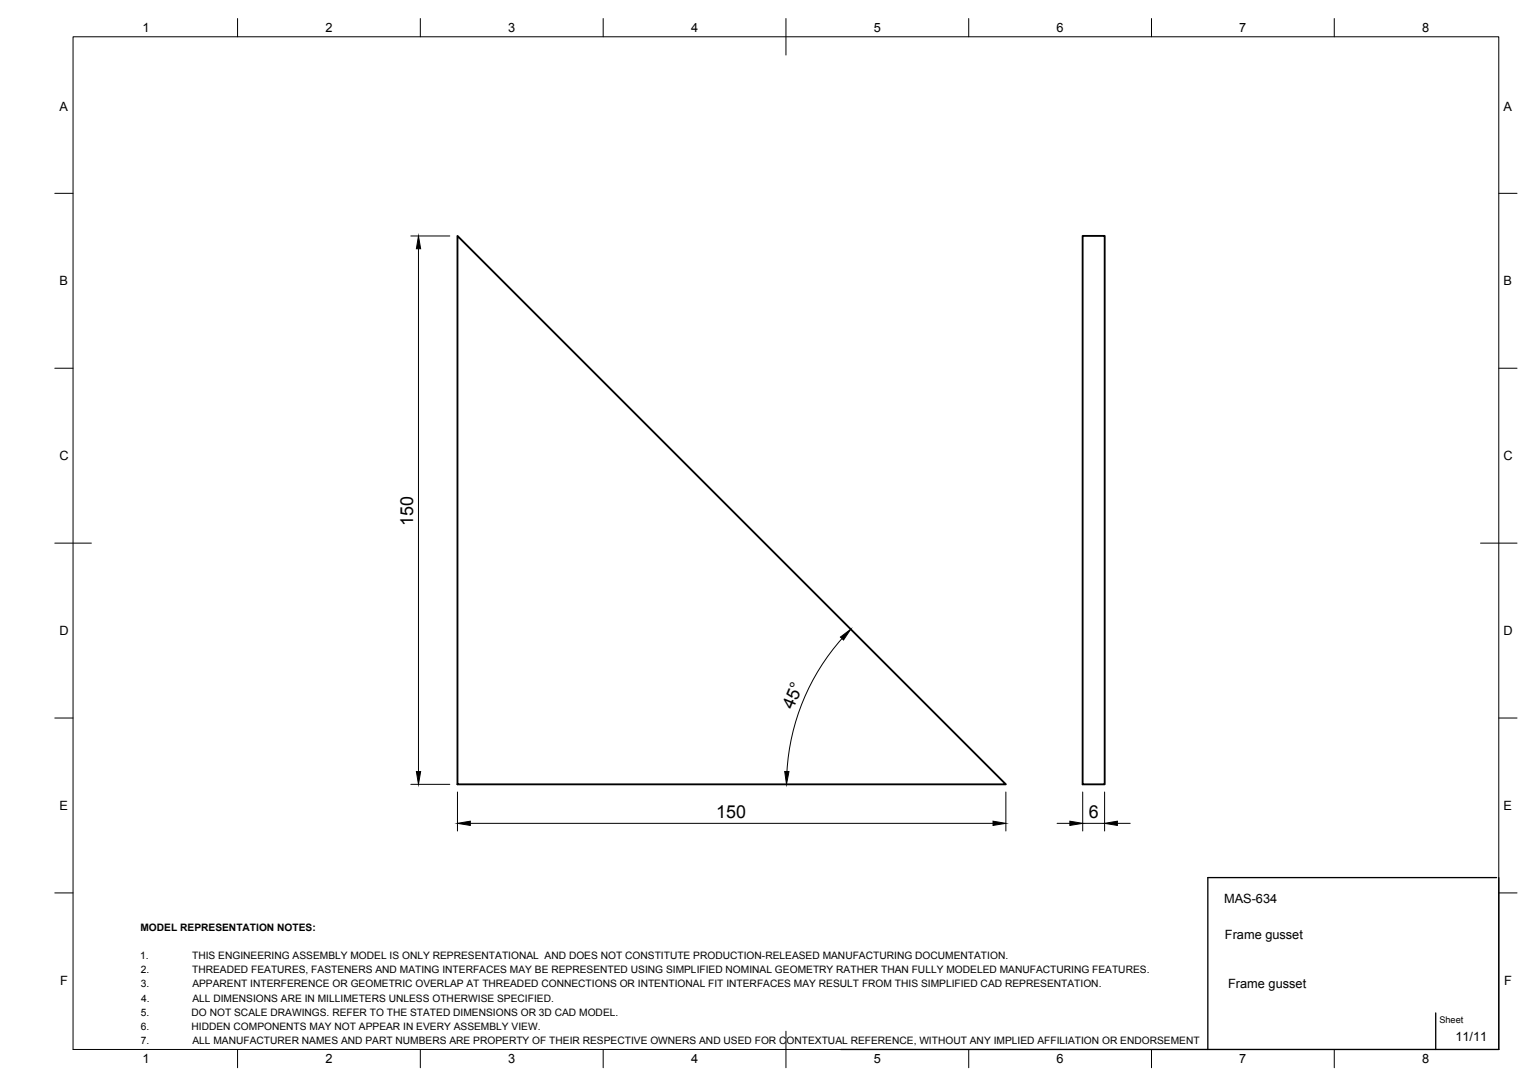
ISO-10303-21;
HEADER;
/* Generated by software containing ST-Developer
 * from STEP Tools, Inc. (www.steptools.com) 
 */

FILE_DESCRIPTION(
/* description */ ('Independent AHU equipment rack. Nominal800x600 frame on1000long40squa
re aluminum posts; two removable notched shelves; welded perimeter/cro
ss rails and rear gussets; two mounting channels; four isolation pads 
and anchor-ready feet. Imported native extrusion library retained and 
cut-length parameters customized per family. Shelf hardware uses model
ed M6 rivet nuts and screws. Weld design, floor anchors and load ratin
g require engineering selection.'),
/* implementation_level */ '2;1');

FILE_NAME(
/* name */ 'Frame gusset.step',
/* time_stamp */ '2026-11-07T19:04:45-08:00',
/* author */ (''),
/* organization */ (''),
/* preprocessor_version */ 'ST-DEVELOPER v20.2',
/* originating_system */ 'Autodesk Translation Framework v15.17.0.0',
/* authorisation */ '');

FILE_SCHEMA (('AUTOMOTIVE_DESIGN { 1 0 10303 214 3 1 1 }'));
ENDSEC;

DATA;
#10=MECHANICAL_DESIGN_GEOMETRIC_PRESENTATION_REPRESENTATION('',(#343),#9777);
#321=SHAPE_REPRESENTATION_RELATIONSHIP('SRR','None',#9865,#332);
#332=ADVANCED_BREP_SHAPE_REPRESENTATION('',(#354),#9774);
#343=STYLED_ITEM('',(#9928),#354);
#354=MANIFOLD_SOLID_BREP('Body1',#3848);
#482=PLANE('',#4211);
#483=PLANE('',#4212);
#484=PLANE('',#4213);
#485=PLANE('',#4214);
#486=PLANE('',#4215);
#626=FACE_OUTER_BOUND('',#870,.T.);
#627=FACE_OUTER_BOUND('',#871,.T.);
#628=FACE_OUTER_BOUND('',#872,.T.);
#629=FACE_OUTER_BOUND('',#873,.T.);
#630=FACE_OUTER_BOUND('',#874,.T.);
#870=EDGE_LOOP('',(#3163,#3164,#3165,#3166));
#871=EDGE_LOOP('',(#3167,#3168,#3169,#3170));
#872=EDGE_LOOP('',(#3171,#3172,#3173,#3174));
#873=EDGE_LOOP('',(#3175,#3176,#3177));
#874=EDGE_LOOP('',(#3178,#3179,#3180));
#1171=LINE('',#6080,#1464);
#1172=LINE('',#6082,#1465);
#1173=LINE('',#6084,#1466);
#1174=LINE('',#6085,#1467);
#1175=LINE('',#6088,#1468);
#1176=LINE('',#6090,#1469);
#1177=LINE('',#6091,#1470);
#1178=LINE('',#6093,#1471);
#1179=LINE('',#6094,#1472);
#1464=VECTOR('',#5050,10.);
#1465=VECTOR('',#5051,10.);
#1466=VECTOR('',#5052,10.);
#1467=VECTOR('',#5053,10.);
#1468=VECTOR('',#5056,10.);
#1469=VECTOR('',#5057,10.);
#1470=VECTOR('',#5058,10.);
#1471=VECTOR('',#5061,10.);
#1472=VECTOR('',#5062,10.);
#1876=VERTEX_POINT('',#6078);
#1877=VERTEX_POINT('',#6079);
#1878=VERTEX_POINT('',#6081);
#1879=VERTEX_POINT('',#6083);
#1880=VERTEX_POINT('',#6087);
#1881=VERTEX_POINT('',#6089);
#2326=EDGE_CURVE('',#1876,#1877,#1171,.T.);
#2327=EDGE_CURVE('',#1877,#1878,#1172,.T.);
#2328=EDGE_CURVE('',#1879,#1878,#1173,.T.);
#2329=EDGE_CURVE('',#1876,#1879,#1174,.T.);
#2330=EDGE_CURVE('',#1880,#1876,#1175,.T.);
#2331=EDGE_CURVE('',#1881,#1879,#1176,.T.);
#2332=EDGE_CURVE('',#1880,#1881,#1177,.T.);
#2333=EDGE_CURVE('',#1877,#1880,#1178,.T.);
#2334=EDGE_CURVE('',#1878,#1881,#1179,.T.);
#3163=ORIENTED_EDGE('',*,*,#2326,.T.);
#3164=ORIENTED_EDGE('',*,*,#2327,.T.);
#3165=ORIENTED_EDGE('',*,*,#2328,.F.);
#3166=ORIENTED_EDGE('',*,*,#2329,.F.);
#3167=ORIENTED_EDGE('',*,*,#2330,.T.);
#3168=ORIENTED_EDGE('',*,*,#2329,.T.);
#3169=ORIENTED_EDGE('',*,*,#2331,.F.);
#3170=ORIENTED_EDGE('',*,*,#2332,.F.);
#3171=ORIENTED_EDGE('',*,*,#2333,.T.);
#3172=ORIENTED_EDGE('',*,*,#2332,.T.);
#3173=ORIENTED_EDGE('',*,*,#2334,.F.);
#3174=ORIENTED_EDGE('',*,*,#2327,.F.);
#3175=ORIENTED_EDGE('',*,*,#2334,.T.);
#3176=ORIENTED_EDGE('',*,*,#2331,.T.);
#3177=ORIENTED_EDGE('',*,*,#2328,.T.);
#3178=ORIENTED_EDGE('',*,*,#2333,.F.);
#3179=ORIENTED_EDGE('',*,*,#2326,.F.);
#3180=ORIENTED_EDGE('',*,*,#2330,.F.);
#3766=ADVANCED_FACE('',(#626),#482,.T.);
#3767=ADVANCED_FACE('',(#627),#483,.T.);
#3768=ADVANCED_FACE('',(#628),#484,.T.);
#3769=ADVANCED_FACE('',(#629),#485,.T.);
#3770=ADVANCED_FACE('',(#630),#486,.F.);
#3848=CLOSED_SHELL('',(#3766,#3767,#3768,#3769,#3770));
#4210=AXIS2_PLACEMENT_3D('',#6076,#5046,#5047);
#4211=AXIS2_PLACEMENT_3D('',#6077,#5048,#5049);
#4212=AXIS2_PLACEMENT_3D('',#6086,#5054,#5055);
#4213=AXIS2_PLACEMENT_3D('',#6092,#5059,#5060);
#4214=AXIS2_PLACEMENT_3D('',#6095,#5063,#5064);
#4215=AXIS2_PLACEMENT_3D('',#6096,#5065,#5066);
#5046=DIRECTION('axis',(0.,0.,1.));
#5047=DIRECTION('refdir',(1.,0.,0.));
#5048=DIRECTION('center_axis',(0.707106781186548,0.707106781186548,0.));
#5049=DIRECTION('ref_axis',(-0.707106781186548,0.707106781186548,0.));
#5050=DIRECTION('',(-0.707106781186547,0.707106781186547,0.));
#5051=DIRECTION('',(0.,0.,1.));
#5052=DIRECTION('',(-0.707106781186547,0.707106781186547,0.));
#5053=DIRECTION('',(0.,0.,1.));
#5054=DIRECTION('center_axis',(0.,-1.,0.));
#5055=DIRECTION('ref_axis',(1.,0.,0.));
#5056=DIRECTION('',(1.,0.,0.));
#5057=DIRECTION('',(1.,0.,0.));
#5058=DIRECTION('',(0.,0.,1.));
#5059=DIRECTION('center_axis',(-1.,0.,0.));
#5060=DIRECTION('ref_axis',(0.,-1.,0.));
#5061=DIRECTION('',(0.,-1.,0.));
#5062=DIRECTION('',(0.,-1.,0.));
#5063=DIRECTION('center_axis',(0.,0.,1.));
#5064=DIRECTION('ref_axis',(1.,0.,0.));
#5065=DIRECTION('center_axis',(0.,0.,1.));
#5066=DIRECTION('ref_axis',(1.,0.,0.));
#6076=CARTESIAN_POINT('',(0.,0.,0.));
#6077=CARTESIAN_POINT('Origin',(150.,0.,0.));
#6078=CARTESIAN_POINT('',(150.,0.,0.));
#6079=CARTESIAN_POINT('',(0.,150.,0.));
#6080=CARTESIAN_POINT('',(150.,0.,0.));
#6081=CARTESIAN_POINT('',(0.,150.,6.));
#6082=CARTESIAN_POINT('',(0.,150.,0.));
#6083=CARTESIAN_POINT('',(150.,0.,6.));
#6084=CARTESIAN_POINT('',(150.,0.,6.));
#6085=CARTESIAN_POINT('',(150.,0.,0.));
#6086=CARTESIAN_POINT('Origin',(0.,0.,0.));
#6087=CARTESIAN_POINT('',(0.,0.,0.));
#6088=CARTESIAN_POINT('',(0.,0.,0.));
#6089=CARTESIAN_POINT('',(0.,0.,6.));
#6090=CARTESIAN_POINT('',(0.,0.,6.));
#6091=CARTESIAN_POINT('',(0.,0.,0.));
#6092=CARTESIAN_POINT('Origin',(0.,150.,0.));
#6093=CARTESIAN_POINT('',(0.,150.,0.));
#6094=CARTESIAN_POINT('',(0.,150.,6.));
#6095=CARTESIAN_POINT('Origin',(75.,75.,6.));
#6096=CARTESIAN_POINT('Origin',(75.,75.,0.));
#9761=UNCERTAINTY_MEASURE_WITH_UNIT(LENGTH_MEASURE(0.01),#9778,
'DISTANCE_ACCURACY_VALUE',
'Maximum model space distance between geometric entities at asserted c
onnectivities');
#9764=UNCERTAINTY_MEASURE_WITH_UNIT(LENGTH_MEASURE(0.01),#9778,
'DISTANCE_ACCURACY_VALUE',
'Maximum model space distance between geometric entities at asserted c
onnectivities');
#9774=(
GEOMETRIC_REPRESENTATION_CONTEXT(3)
GLOBAL_UNCERTAINTY_ASSIGNED_CONTEXT((#9761))
GLOBAL_UNIT_ASSIGNED_CONTEXT((#9778,#9780,#9781))
REPRESENTATION_CONTEXT('','3D')
);
#9777=(
GEOMETRIC_REPRESENTATION_CONTEXT(3)
GLOBAL_UNCERTAINTY_ASSIGNED_CONTEXT((#9764))
GLOBAL_UNIT_ASSIGNED_CONTEXT((#9778,#9780,#9781))
REPRESENTATION_CONTEXT('','3D')
);
#9778=(
LENGTH_UNIT()
NAMED_UNIT(*)
SI_UNIT(.MILLI.,.METRE.)
);
#9780=(
NAMED_UNIT(*)
PLANE_ANGLE_UNIT()
SI_UNIT($,.RADIAN.)
);
#9781=(
NAMED_UNIT(*)
SI_UNIT($,.STERADIAN.)
SOLID_ANGLE_UNIT()
);
#9791=SHAPE_DEFINITION_REPRESENTATION(#9803,#9865);
#9803=PRODUCT_DEFINITION_SHAPE('',$,#9878);
#9865=SHAPE_REPRESENTATION('',(#4210),#9774);
#9868=PRODUCT_DEFINITION_CONTEXT('part definition',#9906,'design');
#9878=PRODUCT_DEFINITION('Frame gusset','Frame gusset',#9890,#9868);
#9890=PRODUCT_DEFINITION_FORMATION('',$,#9917);
#9906=APPLICATION_CONTEXT(
'Core Data for Automotive Mechanical Design Process');
#9907=PRODUCT_CONTEXT('part definition',#9906,'mechanical');
#9917=PRODUCT('Frame gusset','Frame gusset',$,(#9907));
#9928=PRESENTATION_STYLE_ASSIGNMENT((#9939));
#9939=SURFACE_STYLE_USAGE(.BOTH.,#9950);
#9950=SURFACE_SIDE_STYLE('',(#9961));
#9961=SURFACE_STYLE_FILL_AREA(#9972);
#9972=FILL_AREA_STYLE('Gusset gray',(#9983));
#9983=FILL_AREA_STYLE_COLOUR('Gusset gray',#9994);
#9994=COLOUR_RGB('Gusset gray',0.407843137254902,0.447058823529412,0.498039215686275);
ENDSEC;
END-ISO-10303-21;
